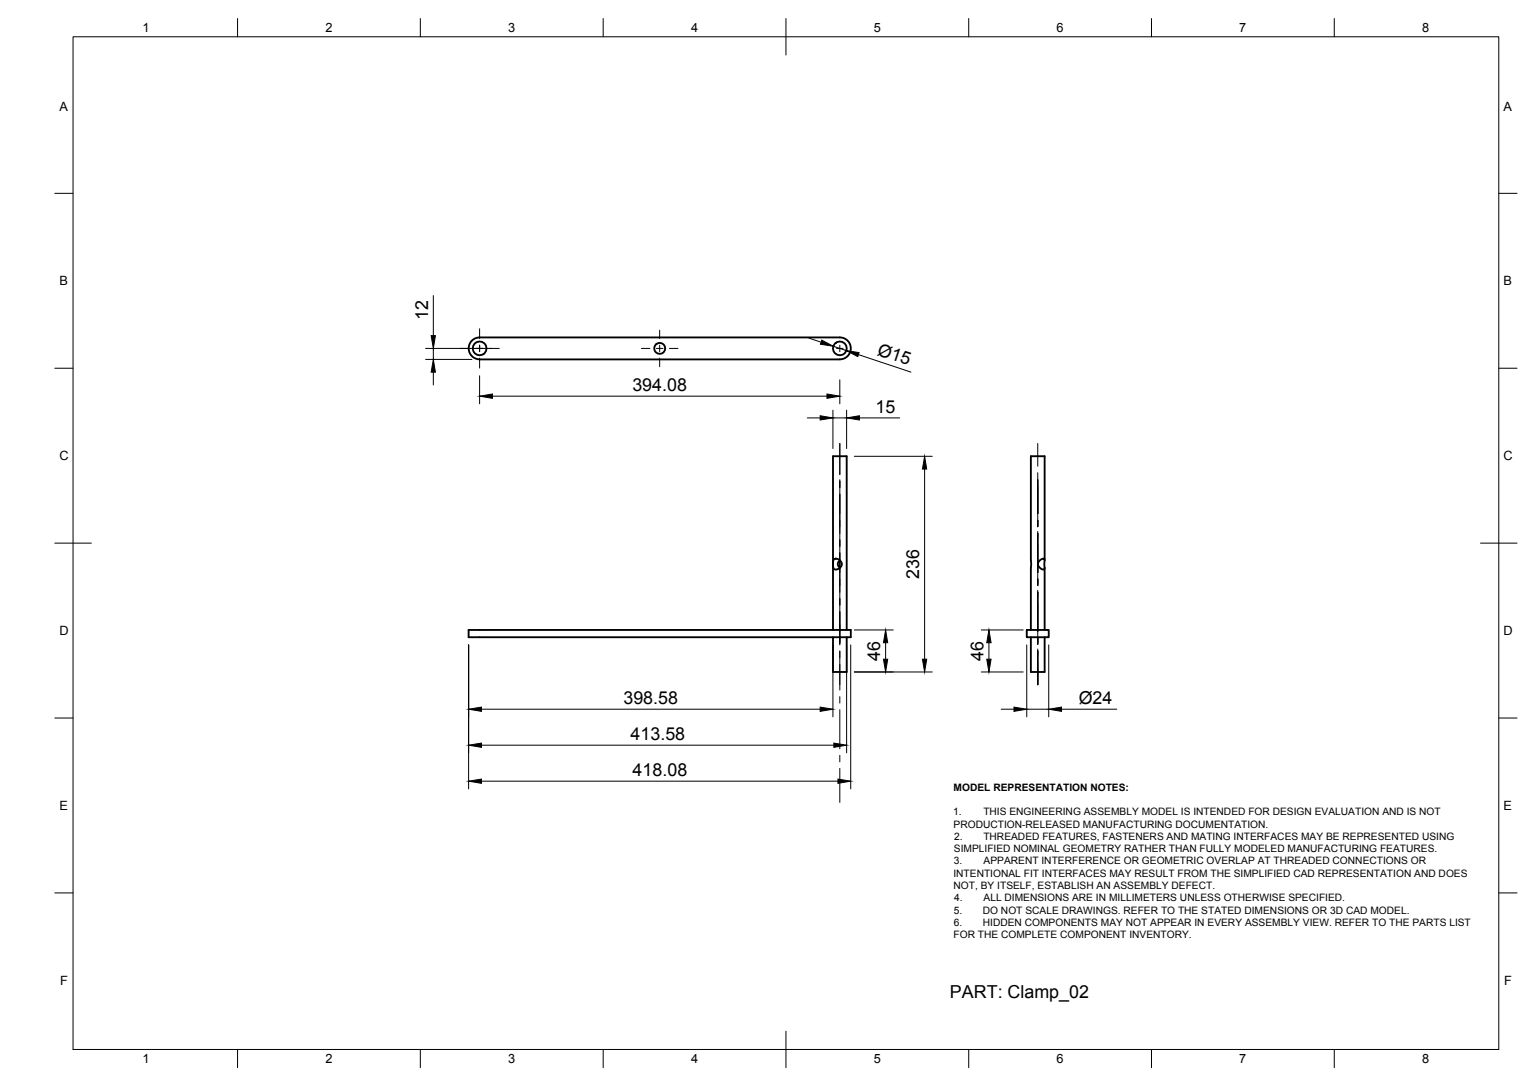
ISO-10303-21;
HEADER;
/* Generated by software containing ST-Developer
 * from STEP Tools, Inc. (www.steptools.com) 
 */

FILE_DESCRIPTION(
/* description */ (''),
/* implementation_level */ '2;1');

FILE_NAME(
/* name */ 'Clamp_02.step',
/* time_stamp */ '2026-10-05T15:35:09-07:00',
/* author */ (''),
/* organization */ (''),
/* preprocessor_version */ 'ST-DEVELOPER v20.2',
/* originating_system */ 'Autodesk Translation Framework v15.15.0.0',
/* authorisation */ '');

FILE_SCHEMA (('AUTOMOTIVE_DESIGN { 1 0 10303 214 3 1 1 }'));
ENDSEC;

DATA;
#10=MECHANICAL_DESIGN_GEOMETRIC_PRESENTATION_REPRESENTATION('',(#547),#74523);
#55=B_SPLINE_CURVE_WITH_KNOTS('',3,(#6168,#6169,#6170,#6171,#6172,#6173,
#6174,#6175,#6176,#6177,#6178,#6179),.UNSPECIFIED.,.F.,.F.,(4,2,2,2,2,4),
(0.,0.123044034193907,0.246088068387815,0.492176136775629,0.730610433663304,
0.969044730550978),.UNSPECIFIED.);
#56=B_SPLINE_CURVE_WITH_KNOTS('',3,(#6180,#6181,#6182,#6183,#6184,#6185,
#6186,#6187,#6188,#6189,#6190,#6191,#6192,#6193,#6194,#6195,#6196,#6197,
#6198,#6199,#6200,#6201,#6202,#6203,#6204,#6205,#6206,#6207,#6208,#6209,
#6210,#6211),.UNSPECIFIED.,.F.,.F.,(4,2,2,2,2,2,2,2,2,2,2,2,2,2,2,4),(0.969044730550978,
1.20747902743865,1.44591332432633,1.69200139271414,1.81504542690805,1.93808946110196,
2.06113349529586,2.18417752948977,2.43026559787759,2.66869989476526,2.90713419165293,
3.14556848854061,3.38400278542828,3.6300908538161,3.75313488801,3.87617892220391),
 .UNSPECIFIED.);
#57=B_SPLINE_CURVE_WITH_KNOTS('',3,(#6215,#6216,#6217,#6218,#6219,#6220,
#6221,#6222,#6223,#6224,#6225,#6226,#6227,#6228,#6229,#6230,#6231,#6232,
#6233,#6234,#6235,#6236),.UNSPECIFIED.,.F.,.F.,(4,2,2,2,2,2,2,2,2,2,4),
(0.969044730550978,1.20747902743865,1.44591332432633,1.69200139271414,1.81504542690805,
1.93808946110196,2.06113349529586,2.18417752948977,2.43026559787759,2.66869989476526,
2.90713419165293),.UNSPECIFIED.);
#58=B_SPLINE_CURVE_WITH_KNOTS('',3,(#6238,#6239,#6240,#6241,#6242,#6243,
#6244,#6245,#6246,#6247,#6248,#6249),.UNSPECIFIED.,.F.,.F.,(4,2,2,2,2,4),
(0.,0.123044034193907,0.246088068387815,0.492176136775629,0.730610433663304,
0.969044730550978),.UNSPECIFIED.);
#59=B_SPLINE_CURVE_WITH_KNOTS('',3,(#6250,#6251,#6252,#6253,#6254,#6255,
#6256,#6257,#6258,#6259,#6260,#6261),.UNSPECIFIED.,.F.,.F.,(4,2,2,2,2,4),
(2.90713419165293,3.14556848854061,3.38400278542828,3.6300908538161,3.75313488801,
3.87617892220391),.UNSPECIFIED.);
#529=SHAPE_REPRESENTATION_RELATIONSHIP('SRR','None',#74562,#538);
#538=ADVANCED_BREP_SHAPE_REPRESENTATION('',(#556),#74518);
#547=STYLED_ITEM('',(#74612),#556);
#556=MANIFOLD_SOLID_BREP('Body1',#4726);
#587=FACE_BOUND('',#924,.T.);
#588=FACE_BOUND('',#925,.T.);
#589=FACE_BOUND('',#926,.T.);
#590=FACE_BOUND('',#928,.T.);
#591=FACE_BOUND('',#929,.T.);
#592=FACE_BOUND('',#930,.T.);
#593=FACE_BOUND('',#934,.T.);
#643=PLANE('',#4968);
#644=PLANE('',#4972);
#645=PLANE('',#4976);
#646=PLANE('',#4978);
#647=PLANE('',#4982);
#648=PLANE('',#4985);
#746=FACE_OUTER_BOUND('',#916,.T.);
#747=FACE_OUTER_BOUND('',#917,.T.);
#748=FACE_OUTER_BOUND('',#918,.T.);
#749=FACE_OUTER_BOUND('',#919,.T.);
#750=FACE_OUTER_BOUND('',#920,.T.);
#751=FACE_OUTER_BOUND('',#921,.T.);
#752=FACE_OUTER_BOUND('',#922,.T.);
#753=FACE_OUTER_BOUND('',#923,.T.);
#754=FACE_OUTER_BOUND('',#927,.T.);
#755=FACE_OUTER_BOUND('',#931,.T.);
#756=FACE_OUTER_BOUND('',#932,.T.);
#757=FACE_OUTER_BOUND('',#933,.T.);
#758=FACE_OUTER_BOUND('',#935,.T.);
#916=EDGE_LOOP('',(#3270,#3271,#3272,#3273));
#917=EDGE_LOOP('',(#3274,#3275,#3276,#3277,#3278,#3279,#3280));
#918=EDGE_LOOP('',(#3281,#3282,#3283,#3284));
#919=EDGE_LOOP('',(#3285,#3286,#3287,#3288));
#920=EDGE_LOOP('',(#3289,#3290,#3291,#3292));
#921=EDGE_LOOP('',(#3293,#3294,#3295,#3296));
#922=EDGE_LOOP('',(#3297,#3298,#3299,#3300));
#923=EDGE_LOOP('',(#3301,#3302,#3303,#3304));
#924=EDGE_LOOP('',(#3305));
#925=EDGE_LOOP('',(#3306));
#926=EDGE_LOOP('',(#3307));
#927=EDGE_LOOP('',(#3308,#3309,#3310,#3311));
#928=EDGE_LOOP('',(#3312));
#929=EDGE_LOOP('',(#3313));
#930=EDGE_LOOP('',(#3314));
#931=EDGE_LOOP('',(#3315,#3316,#3317,#3318));
#932=EDGE_LOOP('',(#3319));
#933=EDGE_LOOP('',(#3320,#3321,#3322,#3323,#3324,#3325,#3326,#3327,#3328));
#934=EDGE_LOOP('',(#3329,#3330));
#935=EDGE_LOOP('',(#3331));
#1114=LINE('',#6163,#1311);
#1115=LINE('',#6213,#1312);
#1116=LINE('',#6266,#1313);
#1117=LINE('',#6271,#1314);
#1118=LINE('',#6273,#1315);
#1119=LINE('',#6275,#1316);
#1120=LINE('',#6276,#1317);
#1121=LINE('',#6282,#1318);
#1122=LINE('',#6285,#1319);
#1123=LINE('',#6287,#1320);
#1124=LINE('',#6288,#1321);
#1125=LINE('',#6301,#1322);
#1126=LINE('',#6304,#1323);
#1127=LINE('',#6306,#1324);
#1311=VECTOR('',#5458,6.00000000000001);
#1312=VECTOR('',#5463,6.);
#1313=VECTOR('',#5468,7.5);
#1314=VECTOR('',#5473,10.);
#1315=VECTOR('',#5474,10.);
#1316=VECTOR('',#5475,10.);
#1317=VECTOR('',#5476,10.);
#1318=VECTOR('',#5483,10.);
#1319=VECTOR('',#5486,10.);
#1320=VECTOR('',#5487,10.);
#1321=VECTOR('',#5488,10.);
#1322=VECTOR('',#5507,7.5);
#1323=VECTOR('',#5512,7.5);
#1324=VECTOR('',#5513,7.5);
#1472=CIRCLE('',#4962,6.00000000000001);
#1473=CIRCLE('',#4963,6.00000000000001);
#1474=CIRCLE('',#4966,7.5);
#1475=CIRCLE('',#4967,7.5);
#1476=CIRCLE('',#4970,12.);
#1477=CIRCLE('',#4971,12.);
#1478=CIRCLE('',#4974,12.);
#1479=CIRCLE('',#4975,12.);
#1480=CIRCLE('',#4977,7.5);
#1481=CIRCLE('',#4979,7.5);
#1482=CIRCLE('',#4981,7.5);
#1483=CIRCLE('',#4984,7.5);
#1626=VERTEX_POINT('',#6160);
#1627=VERTEX_POINT('',#6162);
#1628=VERTEX_POINT('',#6166);
#1629=VERTEX_POINT('',#6167);
#1630=VERTEX_POINT('',#6212);
#1631=VERTEX_POINT('',#6214);
#1632=VERTEX_POINT('',#6237);
#1633=VERTEX_POINT('',#6263);
#1634=VERTEX_POINT('',#6265);
#1635=VERTEX_POINT('',#6269);
#1636=VERTEX_POINT('',#6270);
#1637=VERTEX_POINT('',#6272);
#1638=VERTEX_POINT('',#6274);
#1639=VERTEX_POINT('',#6278);
#1640=VERTEX_POINT('',#6280);
#1641=VERTEX_POINT('',#6284);
#1642=VERTEX_POINT('',#6286);
#1643=VERTEX_POINT('',#6293);
#1644=VERTEX_POINT('',#6296);
#1645=VERTEX_POINT('',#6299);
#1646=VERTEX_POINT('',#6305);
#2336=EDGE_CURVE('',#1626,#1626,#1472,.T.);
#2337=EDGE_CURVE('',#1626,#1627,#1114,.T.);
#2338=EDGE_CURVE('',#1627,#1627,#1473,.T.);
#2339=EDGE_CURVE('',#1628,#1629,#55,.T.);
#2340=EDGE_CURVE('',#1629,#1628,#56,.T.);
#2341=EDGE_CURVE('',#1629,#1630,#1115,.T.);
#2342=EDGE_CURVE('',#1631,#1630,#57,.T.);
#2343=EDGE_CURVE('',#1632,#1631,#58,.T.);
#2344=EDGE_CURVE('',#1630,#1632,#59,.T.);
#2345=EDGE_CURVE('',#1633,#1633,#1474,.T.);
#2346=EDGE_CURVE('',#1633,#1634,#1116,.T.);
#2347=EDGE_CURVE('',#1634,#1634,#1475,.T.);
#2348=EDGE_CURVE('',#1635,#1636,#1117,.T.);
#2349=EDGE_CURVE('',#1636,#1637,#1118,.T.);
#2350=EDGE_CURVE('',#1638,#1637,#1119,.T.);
#2351=EDGE_CURVE('',#1635,#1638,#1120,.T.);
#2352=EDGE_CURVE('',#1639,#1635,#1476,.T.);
#2353=EDGE_CURVE('',#1640,#1638,#1477,.T.);
#2354=EDGE_CURVE('',#1639,#1640,#1121,.T.);
#2355=EDGE_CURVE('',#1641,#1639,#1122,.T.);
#2356=EDGE_CURVE('',#1642,#1640,#1123,.T.);
#2357=EDGE_CURVE('',#1641,#1642,#1124,.T.);
#2358=EDGE_CURVE('',#1636,#1641,#1478,.T.);
#2359=EDGE_CURVE('',#1637,#1642,#1479,.T.);
#2360=EDGE_CURVE('',#1643,#1643,#1480,.T.);
#2361=EDGE_CURVE('',#1644,#1644,#1481,.T.);
#2362=EDGE_CURVE('',#1645,#1645,#1482,.T.);
#2363=EDGE_CURVE('',#1645,#1644,#1125,.T.);
#2364=EDGE_CURVE('',#1643,#1630,#1126,.T.);
#2365=EDGE_CURVE('',#1631,#1646,#1127,.T.);
#2366=EDGE_CURVE('',#1646,#1646,#1483,.T.);
#3270=ORIENTED_EDGE('',*,*,#2336,.F.);
#3271=ORIENTED_EDGE('',*,*,#2337,.T.);
#3272=ORIENTED_EDGE('',*,*,#2338,.F.);
#3273=ORIENTED_EDGE('',*,*,#2337,.F.);
#3274=ORIENTED_EDGE('',*,*,#2339,.F.);
#3275=ORIENTED_EDGE('',*,*,#2340,.F.);
#3276=ORIENTED_EDGE('',*,*,#2341,.T.);
#3277=ORIENTED_EDGE('',*,*,#2342,.F.);
#3278=ORIENTED_EDGE('',*,*,#2343,.F.);
#3279=ORIENTED_EDGE('',*,*,#2344,.F.);
#3280=ORIENTED_EDGE('',*,*,#2341,.F.);
#3281=ORIENTED_EDGE('',*,*,#2345,.T.);
#3282=ORIENTED_EDGE('',*,*,#2346,.T.);
#3283=ORIENTED_EDGE('',*,*,#2347,.F.);
#3284=ORIENTED_EDGE('',*,*,#2346,.F.);
#3285=ORIENTED_EDGE('',*,*,#2348,.T.);
#3286=ORIENTED_EDGE('',*,*,#2349,.T.);
#3287=ORIENTED_EDGE('',*,*,#2350,.F.);
#3288=ORIENTED_EDGE('',*,*,#2351,.F.);
#3289=ORIENTED_EDGE('',*,*,#2352,.T.);
#3290=ORIENTED_EDGE('',*,*,#2351,.T.);
#3291=ORIENTED_EDGE('',*,*,#2353,.F.);
#3292=ORIENTED_EDGE('',*,*,#2354,.F.);
#3293=ORIENTED_EDGE('',*,*,#2355,.T.);
#3294=ORIENTED_EDGE('',*,*,#2354,.T.);
#3295=ORIENTED_EDGE('',*,*,#2356,.F.);
#3296=ORIENTED_EDGE('',*,*,#2357,.F.);
#3297=ORIENTED_EDGE('',*,*,#2358,.T.);
#3298=ORIENTED_EDGE('',*,*,#2357,.T.);
#3299=ORIENTED_EDGE('',*,*,#2359,.F.);
#3300=ORIENTED_EDGE('',*,*,#2349,.F.);
#3301=ORIENTED_EDGE('',*,*,#2359,.T.);
#3302=ORIENTED_EDGE('',*,*,#2356,.T.);
#3303=ORIENTED_EDGE('',*,*,#2353,.T.);
#3304=ORIENTED_EDGE('',*,*,#2350,.T.);
#3305=ORIENTED_EDGE('',*,*,#2336,.T.);
#3306=ORIENTED_EDGE('',*,*,#2360,.F.);
#3307=ORIENTED_EDGE('',*,*,#2347,.T.);
#3308=ORIENTED_EDGE('',*,*,#2358,.F.);
#3309=ORIENTED_EDGE('',*,*,#2348,.F.);
#3310=ORIENTED_EDGE('',*,*,#2352,.F.);
#3311=ORIENTED_EDGE('',*,*,#2355,.F.);
#3312=ORIENTED_EDGE('',*,*,#2338,.T.);
#3313=ORIENTED_EDGE('',*,*,#2361,.F.);
#3314=ORIENTED_EDGE('',*,*,#2345,.F.);
#3315=ORIENTED_EDGE('',*,*,#2362,.T.);
#3316=ORIENTED_EDGE('',*,*,#2363,.T.);
#3317=ORIENTED_EDGE('',*,*,#2361,.T.);
#3318=ORIENTED_EDGE('',*,*,#2363,.F.);
#3319=ORIENTED_EDGE('',*,*,#2362,.F.);
#3320=ORIENTED_EDGE('',*,*,#2360,.T.);
#3321=ORIENTED_EDGE('',*,*,#2364,.T.);
#3322=ORIENTED_EDGE('',*,*,#2344,.T.);
#3323=ORIENTED_EDGE('',*,*,#2343,.T.);
#3324=ORIENTED_EDGE('',*,*,#2365,.T.);
#3325=ORIENTED_EDGE('',*,*,#2366,.T.);
#3326=ORIENTED_EDGE('',*,*,#2365,.F.);
#3327=ORIENTED_EDGE('',*,*,#2342,.T.);
#3328=ORIENTED_EDGE('',*,*,#2364,.F.);
#3329=ORIENTED_EDGE('',*,*,#2339,.T.);
#3330=ORIENTED_EDGE('',*,*,#2340,.T.);
#3331=ORIENTED_EDGE('',*,*,#2366,.F.);
#4544=CYLINDRICAL_SURFACE('',#4961,6.00000000000001);
#4545=CYLINDRICAL_SURFACE('',#4964,6.);
#4546=CYLINDRICAL_SURFACE('',#4965,7.5);
#4547=CYLINDRICAL_SURFACE('',#4969,12.);
#4548=CYLINDRICAL_SURFACE('',#4973,12.);
#4549=CYLINDRICAL_SURFACE('',#4980,7.5);
#4550=CYLINDRICAL_SURFACE('',#4983,7.5);
#4642=ADVANCED_FACE('',(#746),#4544,.F.);
#4643=ADVANCED_FACE('',(#747),#4545,.F.);
#4644=ADVANCED_FACE('',(#748),#4546,.F.);
#4645=ADVANCED_FACE('',(#749),#643,.T.);
#4646=ADVANCED_FACE('',(#750),#4547,.T.);
#4647=ADVANCED_FACE('',(#751),#644,.T.);
#4648=ADVANCED_FACE('',(#752),#4548,.T.);
#4649=ADVANCED_FACE('',(#753,#587,#588,#589),#645,.T.);
#4650=ADVANCED_FACE('',(#754,#590,#591,#592),#646,.F.);
#4651=ADVANCED_FACE('',(#755),#4549,.T.);
#4652=ADVANCED_FACE('',(#756),#647,.T.);
#4653=ADVANCED_FACE('',(#757,#593),#4550,.T.);
#4654=ADVANCED_FACE('',(#758),#648,.F.);
#4726=CLOSED_SHELL('',(#4642,#4643,#4644,#4645,#4646,#4647,#4648,#4649,
#4650,#4651,#4652,#4653,#4654));
#4960=AXIS2_PLACEMENT_3D('',#6158,#5452,#5453);
#4961=AXIS2_PLACEMENT_3D('',#6159,#5454,#5455);
#4962=AXIS2_PLACEMENT_3D('',#6161,#5456,#5457);
#4963=AXIS2_PLACEMENT_3D('',#6164,#5459,#5460);
#4964=AXIS2_PLACEMENT_3D('',#6165,#5461,#5462);
#4965=AXIS2_PLACEMENT_3D('',#6262,#5464,#5465);
#4966=AXIS2_PLACEMENT_3D('',#6264,#5466,#5467);
#4967=AXIS2_PLACEMENT_3D('',#6267,#5469,#5470);
#4968=AXIS2_PLACEMENT_3D('',#6268,#5471,#5472);
#4969=AXIS2_PLACEMENT_3D('',#6277,#5477,#5478);
#4970=AXIS2_PLACEMENT_3D('',#6279,#5479,#5480);
#4971=AXIS2_PLACEMENT_3D('',#6281,#5481,#5482);
#4972=AXIS2_PLACEMENT_3D('',#6283,#5484,#5485);
#4973=AXIS2_PLACEMENT_3D('',#6289,#5489,#5490);
#4974=AXIS2_PLACEMENT_3D('',#6290,#5491,#5492);
#4975=AXIS2_PLACEMENT_3D('',#6291,#5493,#5494);
#4976=AXIS2_PLACEMENT_3D('',#6292,#5495,#5496);
#4977=AXIS2_PLACEMENT_3D('',#6294,#5497,#5498);
#4978=AXIS2_PLACEMENT_3D('',#6295,#5499,#5500);
#4979=AXIS2_PLACEMENT_3D('',#6297,#5501,#5502);
#4980=AXIS2_PLACEMENT_3D('',#6298,#5503,#5504);
#4981=AXIS2_PLACEMENT_3D('',#6300,#5505,#5506);
#4982=AXIS2_PLACEMENT_3D('',#6302,#5508,#5509);
#4983=AXIS2_PLACEMENT_3D('',#6303,#5510,#5511);
#4984=AXIS2_PLACEMENT_3D('',#6307,#5514,#5515);
#4985=AXIS2_PLACEMENT_3D('',#6308,#5516,#5517);
#5452=DIRECTION('axis',(0.,0.,1.));
#5453=DIRECTION('refdir',(1.,0.,0.));
#5454=DIRECTION('center_axis',(0.,-1.,0.));
#5455=DIRECTION('ref_axis',(1.,0.,0.));
#5456=DIRECTION('center_axis',(0.,-1.,0.));
#5457=DIRECTION('ref_axis',(1.,0.,0.));
#5458=DIRECTION('',(0.,-1.,0.));
#5459=DIRECTION('center_axis',(0.,1.,0.));
#5460=DIRECTION('ref_axis',(1.,0.,0.));
#5461=DIRECTION('center_axis',(-1.,0.,0.));
#5462=DIRECTION('ref_axis',(0.,1.,0.));
#5463=DIRECTION('',(-1.,0.,0.));
#5464=DIRECTION('center_axis',(0.,1.,0.));
#5465=DIRECTION('ref_axis',(1.,0.,0.));
#5466=DIRECTION('center_axis',(0.,-1.,0.));
#5467=DIRECTION('ref_axis',(1.,0.,0.));
#5468=DIRECTION('',(0.,1.,0.));
#5469=DIRECTION('center_axis',(0.,-1.,0.));
#5470=DIRECTION('ref_axis',(1.,0.,0.));
#5471=DIRECTION('center_axis',(-0.812015371342714,0.,0.583636048152575));
#5472=DIRECTION('ref_axis',(0.583636048152575,0.,0.812015371342714));
#5473=DIRECTION('',(0.583636048152575,0.,0.812015371342714));
#5474=DIRECTION('',(0.,1.,0.));
#5475=DIRECTION('',(0.583636048152575,0.,0.812015371342714));
#5476=DIRECTION('',(0.,1.,0.));
#5477=DIRECTION('center_axis',(0.,1.,0.));
#5478=DIRECTION('ref_axis',(0.812015371342714,0.,-0.583636048152574));
#5479=DIRECTION('center_axis',(0.,1.,0.));
#5480=DIRECTION('ref_axis',(0.812015371342714,0.,-0.583636048152574));
#5481=DIRECTION('center_axis',(0.,1.,0.));
#5482=DIRECTION('ref_axis',(0.812015371342714,0.,-0.583636048152574));
#5483=DIRECTION('',(0.,1.,0.));
#5484=DIRECTION('center_axis',(0.812015371342714,0.,-0.583636048152575));
#5485=DIRECTION('ref_axis',(-0.583636048152575,0.,-0.812015371342714));
#5486=DIRECTION('',(-0.583636048152575,0.,-0.812015371342714));
#5487=DIRECTION('',(-0.583636048152575,0.,-0.812015371342714));
#5488=DIRECTION('',(0.,1.,0.));
#5489=DIRECTION('center_axis',(0.,1.,0.));
#5490=DIRECTION('ref_axis',(-0.812015371342714,0.,0.583636048152574));
#5491=DIRECTION('center_axis',(0.,1.,0.));
#5492=DIRECTION('ref_axis',(-0.812015371342714,0.,0.583636048152574));
#5493=DIRECTION('center_axis',(0.,1.,0.));
#5494=DIRECTION('ref_axis',(-0.812015371342714,0.,0.583636048152574));
#5495=DIRECTION('center_axis',(0.,1.,0.));
#5496=DIRECTION('ref_axis',(1.,0.,0.));
#5497=DIRECTION('center_axis',(0.,1.,0.));
#5498=DIRECTION('ref_axis',(1.,0.,2.44929359829471E-16));
#5499=DIRECTION('center_axis',(0.,1.,0.));
#5500=DIRECTION('ref_axis',(1.,0.,0.));
#5501=DIRECTION('center_axis',(0.,-1.,0.));
#5502=DIRECTION('ref_axis',(1.,0.,2.44929359829471E-16));
#5503=DIRECTION('center_axis',(-3.66477378287572E-33,-1.,2.99251489117293E-17));
#5504=DIRECTION('ref_axis',(1.,3.66477378287573E-33,2.44929359829471E-16));
#5505=DIRECTION('center_axis',(3.66477378287572E-33,1.,-2.99251489117293E-17));
#5506=DIRECTION('ref_axis',(1.,3.66477378287573E-33,2.44929359829471E-16));
#5507=DIRECTION('',(3.66477378287572E-33,1.,-2.99251489117293E-17));
#5508=DIRECTION('center_axis',(-3.66477378287572E-33,-1.,2.99251489117293E-17));
#5509=DIRECTION('ref_axis',(1.,3.66477378287573E-33,2.44929359829471E-16));
#5510=DIRECTION('center_axis',(-3.66477378287572E-33,-1.,2.99251489117293E-17));
#5511=DIRECTION('ref_axis',(1.,3.66477378287573E-33,2.44929359829471E-16));
#5512=DIRECTION('',(3.66477378287572E-33,1.,-2.99251489117293E-17));
#5513=DIRECTION('',(3.66477378287572E-33,1.,-2.99251489117293E-17));
#5514=DIRECTION('center_axis',(-3.66477378287572E-33,-1.,2.99251489117293E-17));
#5515=DIRECTION('ref_axis',(1.,3.66477378287573E-33,2.44929359829471E-16));
#5516=DIRECTION('center_axis',(-3.66477378287572E-33,-1.,2.99251489117293E-17));
#5517=DIRECTION('ref_axis',(1.,3.66477378287573E-33,2.44929359829471E-16));
#6158=CARTESIAN_POINT('',(0.,0.,0.));
#6159=CARTESIAN_POINT('Origin',(60.231676812499,-95.,175.));
#6160=CARTESIAN_POINT('',(54.231676812499,-72.,175.));
#6161=CARTESIAN_POINT('Origin',(60.231676812499,-72.,175.));
#6162=CARTESIAN_POINT('',(54.231676812499,-80.,175.));
#6163=CARTESIAN_POINT('',(54.231676812499,-95.,175.));
#6164=CARTESIAN_POINT('Origin',(60.231676812499,-80.,175.));
#6165=CARTESIAN_POINT('Origin',(185.231676812499,0.,335.));
#6166=CARTESIAN_POINT('',(179.731676812499,2.46330733588707E-15,329.));
#6167=CARTESIAN_POINT('',(182.731676812499,-6.,335.));
#6168=CARTESIAN_POINT('Ctrl Pts',(179.731676812499,-1.38777878078145E-16,
329.));
#6169=CARTESIAN_POINT('Ctrl Pts',(179.731676812499,-0.410146780646358,329.));
#6170=CARTESIAN_POINT('Ctrl Pts',(179.789372806578,-0.816861849349989,329.042276815307));
#6171=CARTESIAN_POINT('Ctrl Pts',(179.994045571984,-1.60462674459781,329.204579222783));
#6172=CARTESIAN_POINT('Ctrl Pts',(180.139940991557,-1.98596758305952,329.324554046353));
#6173=CARTESIAN_POINT('Ctrl Pts',(180.642335947217,-3.07201535485507,329.786388864399));
#6174=CARTESIAN_POINT('Ctrl Pts',(181.058329790287,-3.7207625323499,330.235481158111));
#6175=CARTESIAN_POINT('Ctrl Pts',(181.763206112437,-4.74828751391861,331.26300613968));
#6176=CARTESIAN_POINT('Ctrl Pts',(182.110324034524,-5.20624497170395,331.912343858094));
#6177=CARTESIAN_POINT('Ctrl Pts',(182.596018078742,-5.8328999714949,333.382629157599));
#6178=CARTESIAN_POINT('Ctrl Pts',(182.731676812499,-6.00000000000001,334.205219010374));
#6179=CARTESIAN_POINT('Ctrl Pts',(182.731676812499,-6.00000000000001,335.));
#6180=CARTESIAN_POINT('Ctrl Pts',(182.731676812499,-6.,335.));
#6181=CARTESIAN_POINT('Ctrl Pts',(182.731676812499,-6.,335.794780989626));
#6182=CARTESIAN_POINT('Ctrl Pts',(182.596018078742,-5.8328999714949,336.617370842401));
#6183=CARTESIAN_POINT('Ctrl Pts',(182.110324034524,-5.20624497170395,338.087656141906));
#6184=CARTESIAN_POINT('Ctrl Pts',(181.763206112437,-4.74828751391861,338.73699386032));
#6185=CARTESIAN_POINT('Ctrl Pts',(181.058329790287,-3.7207625323499,339.764518841889));
#6186=CARTESIAN_POINT('Ctrl Pts',(180.642335947217,-3.07201535485507,340.213611135601));
#6187=CARTESIAN_POINT('Ctrl Pts',(180.139940991557,-1.98596758305952,340.675445953647));
#6188=CARTESIAN_POINT('Ctrl Pts',(179.994045571984,-1.60462674459781,340.795420777217));
#6189=CARTESIAN_POINT('Ctrl Pts',(179.789372806578,-0.816861849349989,340.957723184693));
#6190=CARTESIAN_POINT('Ctrl Pts',(179.731676812499,-0.410146780646358,341.));
#6191=CARTESIAN_POINT('Ctrl Pts',(179.731676812499,0.410146780646357,341.));
#6192=CARTESIAN_POINT('Ctrl Pts',(179.789372806578,0.816861849350014,340.957723184693));
#6193=CARTESIAN_POINT('Ctrl Pts',(179.994045571984,1.60462674459784,340.795420777217));
#6194=CARTESIAN_POINT('Ctrl Pts',(180.139940991557,1.9859675830595,340.675445953647));
#6195=CARTESIAN_POINT('Ctrl Pts',(180.642335947218,3.07201535485506,340.213611135601));
#6196=CARTESIAN_POINT('Ctrl Pts',(181.058329790287,3.7207625323499,339.764518841889));
#6197=CARTESIAN_POINT('Ctrl Pts',(181.763206112437,4.74828751391861,338.73699386032));
#6198=CARTESIAN_POINT('Ctrl Pts',(182.110324034524,5.20624497170395,338.087656141906));
#6199=CARTESIAN_POINT('Ctrl Pts',(182.596018078742,5.8328999714949,336.617370842401));
#6200=CARTESIAN_POINT('Ctrl Pts',(182.731676812499,6.,335.794780989626));
#6201=CARTESIAN_POINT('Ctrl Pts',(182.731676812499,6.,334.205219010374));
#6202=CARTESIAN_POINT('Ctrl Pts',(182.596018078742,5.8328999714949,333.382629157599));
#6203=CARTESIAN_POINT('Ctrl Pts',(182.110324034524,5.20624497170395,331.912343858094));
#6204=CARTESIAN_POINT('Ctrl Pts',(181.763206112437,4.74828751391861,331.26300613968));
#6205=CARTESIAN_POINT('Ctrl Pts',(181.058329790287,3.7207625323499,330.235481158111));
#6206=CARTESIAN_POINT('Ctrl Pts',(180.642335947218,3.07201535485506,329.786388864399));
#6207=CARTESIAN_POINT('Ctrl Pts',(180.139940991557,1.9859675830595,329.324554046353));
#6208=CARTESIAN_POINT('Ctrl Pts',(179.994045571984,1.60462674459784,329.204579222783));
#6209=CARTESIAN_POINT('Ctrl Pts',(179.789372806578,0.816861849350014,329.042276815307));
#6210=CARTESIAN_POINT('Ctrl Pts',(179.731676812499,0.410146780646354,329.));
#6211=CARTESIAN_POINT('Ctrl Pts',(179.731676812499,-2.67147415300428E-15,
329.));
#6212=CARTESIAN_POINT('',(167.731676812499,-6.,335.));
#6213=CARTESIAN_POINT('',(185.231676812499,-6.,335.));
#6214=CARTESIAN_POINT('',(167.731676812499,6.,335.));
#6215=CARTESIAN_POINT('Ctrl Pts',(167.731676812499,6.,335.));
#6216=CARTESIAN_POINT('Ctrl Pts',(167.731676812499,6.,335.794780989625));
#6217=CARTESIAN_POINT('Ctrl Pts',(167.867335546256,5.8328999714949,336.617370842401));
#6218=CARTESIAN_POINT('Ctrl Pts',(168.353029590474,5.20624497170395,338.087656141906));
#6219=CARTESIAN_POINT('Ctrl Pts',(168.700147512561,4.74828751391861,338.73699386032));
#6220=CARTESIAN_POINT('Ctrl Pts',(169.405023834711,3.7207625323499,339.764518841889));
#6221=CARTESIAN_POINT('Ctrl Pts',(169.821017677781,3.07201535485507,340.213611135601));
#6222=CARTESIAN_POINT('Ctrl Pts',(170.323412633441,1.98596758305952,340.675445953647));
#6223=CARTESIAN_POINT('Ctrl Pts',(170.469308053014,1.60462674459781,340.795420777217));
#6224=CARTESIAN_POINT('Ctrl Pts',(170.67398081842,0.81686184934999,340.957723184693));
#6225=CARTESIAN_POINT('Ctrl Pts',(170.731676812499,0.410146780646358,341.));
#6226=CARTESIAN_POINT('Ctrl Pts',(170.731676812499,-0.410146780646357,341.));
#6227=CARTESIAN_POINT('Ctrl Pts',(170.67398081842,-0.816861849349986,340.957723184693));
#6228=CARTESIAN_POINT('Ctrl Pts',(170.469308053014,-1.60462674459781,340.795420777217));
#6229=CARTESIAN_POINT('Ctrl Pts',(170.323412633441,-1.98596758305952,340.675445953647));
#6230=CARTESIAN_POINT('Ctrl Pts',(169.821017677781,-3.07201535485507,340.213611135601));
#6231=CARTESIAN_POINT('Ctrl Pts',(169.405023834711,-3.7207625323499,339.764518841889));
#6232=CARTESIAN_POINT('Ctrl Pts',(168.700147512561,-4.74828751391861,338.73699386032));
#6233=CARTESIAN_POINT('Ctrl Pts',(168.353029590474,-5.20624497170395,338.087656141906));
#6234=CARTESIAN_POINT('Ctrl Pts',(167.867335546256,-5.8328999714949,336.617370842401));
#6235=CARTESIAN_POINT('Ctrl Pts',(167.731676812499,-6.,335.794780989626));
#6236=CARTESIAN_POINT('Ctrl Pts',(167.731676812499,-6.,335.));
#6237=CARTESIAN_POINT('',(170.731676812499,5.89805981832114E-16,329.));
#6238=CARTESIAN_POINT('Ctrl Pts',(170.731676812499,1.2490009027033E-15,
329.));
#6239=CARTESIAN_POINT('Ctrl Pts',(170.731676812499,0.410146780646359,329.));
#6240=CARTESIAN_POINT('Ctrl Pts',(170.67398081842,0.816861849349989,329.042276815307));
#6241=CARTESIAN_POINT('Ctrl Pts',(170.469308053014,1.60462674459781,329.204579222783));
#6242=CARTESIAN_POINT('Ctrl Pts',(170.323412633441,1.98596758305952,329.324554046353));
#6243=CARTESIAN_POINT('Ctrl Pts',(169.821017677781,3.07201535485507,329.786388864399));
#6244=CARTESIAN_POINT('Ctrl Pts',(169.405023834711,3.7207625323499,330.235481158111));
#6245=CARTESIAN_POINT('Ctrl Pts',(168.700147512561,4.74828751391861,331.26300613968));
#6246=CARTESIAN_POINT('Ctrl Pts',(168.353029590474,5.20624497170395,331.912343858094));
#6247=CARTESIAN_POINT('Ctrl Pts',(167.867335546256,5.8328999714949,333.382629157599));
#6248=CARTESIAN_POINT('Ctrl Pts',(167.731676812499,6.,334.205219010374));
#6249=CARTESIAN_POINT('Ctrl Pts',(167.731676812499,6.,335.));
#6250=CARTESIAN_POINT('Ctrl Pts',(167.731676812499,-6.,335.));
#6251=CARTESIAN_POINT('Ctrl Pts',(167.731676812499,-6.,334.205219010374));
#6252=CARTESIAN_POINT('Ctrl Pts',(167.867335546256,-5.8328999714949,333.382629157599));
#6253=CARTESIAN_POINT('Ctrl Pts',(168.353029590474,-5.20624497170395,331.912343858094));
#6254=CARTESIAN_POINT('Ctrl Pts',(168.700147512561,-4.74828751391861,331.26300613968));
#6255=CARTESIAN_POINT('Ctrl Pts',(169.405023834711,-3.7207625323499,330.235481158111));
#6256=CARTESIAN_POINT('Ctrl Pts',(169.821017677781,-3.07201535485506,329.786388864399));
#6257=CARTESIAN_POINT('Ctrl Pts',(170.323412633441,-1.98596758305952,329.324554046353));
#6258=CARTESIAN_POINT('Ctrl Pts',(170.469308053014,-1.60462674459781,329.204579222783));
#6259=CARTESIAN_POINT('Ctrl Pts',(170.67398081842,-0.816861849349986,329.042276815307));
#6260=CARTESIAN_POINT('Ctrl Pts',(170.731676812499,-0.410146780646357,329.));
#6261=CARTESIAN_POINT('Ctrl Pts',(170.731676812499,-1.79550893470375E-16,
329.));
#6262=CARTESIAN_POINT('Origin',(-54.7683231875009,-80.,15.));
#6263=CARTESIAN_POINT('',(-62.2683231875009,-80.,15.));
#6264=CARTESIAN_POINT('Origin',(-54.7683231875009,-80.,15.));
#6265=CARTESIAN_POINT('',(-62.2683231875009,-72.,15.));
#6266=CARTESIAN_POINT('',(-62.2683231875009,-80.,15.));
#6267=CARTESIAN_POINT('Origin',(-54.7683231875009,-72.,15.));
#6268=CARTESIAN_POINT('Origin',(-64.5125076436135,-80.,22.0036325778309));
#6269=CARTESIAN_POINT('',(-64.5125076436135,-80.,22.0036325778309));
#6270=CARTESIAN_POINT('',(165.487492356386,-80.,342.003632577831));
#6271=CARTESIAN_POINT('',(-64.5125076436135,-80.,22.0036325778309));
#6272=CARTESIAN_POINT('',(165.487492356386,-72.,342.003632577831));
#6273=CARTESIAN_POINT('',(165.487492356386,-80.,342.003632577831));
#6274=CARTESIAN_POINT('',(-64.5125076436135,-72.,22.0036325778309));
#6275=CARTESIAN_POINT('',(-64.5125076436135,-72.,22.0036325778309));
#6276=CARTESIAN_POINT('',(-64.5125076436135,-80.,22.0036325778309));
#6277=CARTESIAN_POINT('Origin',(-54.7683231875009,-80.,15.));
#6278=CARTESIAN_POINT('',(-45.0241387313884,-80.,7.99636742216912));
#6279=CARTESIAN_POINT('Origin',(-54.7683231875009,-80.,15.));
#6280=CARTESIAN_POINT('',(-45.0241387313884,-72.,7.99636742216912));
#6281=CARTESIAN_POINT('Origin',(-54.7683231875009,-72.,15.));
#6282=CARTESIAN_POINT('',(-45.0241387313884,-80.,7.99636742216912));
#6283=CARTESIAN_POINT('Origin',(184.975861268612,-80.,327.996367422169));
#6284=CARTESIAN_POINT('',(184.975861268612,-80.,327.996367422169));
#6285=CARTESIAN_POINT('',(184.975861268612,-80.,327.996367422169));
#6286=CARTESIAN_POINT('',(184.975861268612,-72.,327.996367422169));
#6287=CARTESIAN_POINT('',(184.975861268612,-72.,327.996367422169));
#6288=CARTESIAN_POINT('',(184.975861268612,-80.,327.996367422169));
#6289=CARTESIAN_POINT('Origin',(175.231676812499,-80.,335.));
#6290=CARTESIAN_POINT('Origin',(175.231676812499,-80.,335.));
#6291=CARTESIAN_POINT('Origin',(175.231676812499,-72.,335.));
#6292=CARTESIAN_POINT('Origin',(60.231676812499,-72.,175.));
#6293=CARTESIAN_POINT('',(167.731676812499,-72.,335.));
#6294=CARTESIAN_POINT('Origin',(175.231676812499,-72.,335.));
#6295=CARTESIAN_POINT('Origin',(60.231676812499,-80.,175.));
#6296=CARTESIAN_POINT('',(167.731676812499,-80.,335.));
#6297=CARTESIAN_POINT('Origin',(175.231676812499,-80.,335.));
#6298=CARTESIAN_POINT('Origin',(175.231676812499,4.78802382587669E-15,335.));
#6299=CARTESIAN_POINT('',(167.731676812499,-118.,335.));
#6300=CARTESIAN_POINT('Origin',(175.231676812499,-118.,335.));
#6301=CARTESIAN_POINT('',(167.731676812499,4.78802382587669E-15,335.));
#6302=CARTESIAN_POINT('Origin',(175.231676812499,-118.,335.));
#6303=CARTESIAN_POINT('Origin',(175.231676812499,4.78802382587669E-15,335.));
#6304=CARTESIAN_POINT('',(167.731676812499,4.78802382587669E-15,335.));
#6305=CARTESIAN_POINT('',(167.731676812499,118.,335.));
#6306=CARTESIAN_POINT('',(167.731676812499,4.78802382587669E-15,335.));
#6307=CARTESIAN_POINT('Origin',(175.231676812499,118.,335.));
#6308=CARTESIAN_POINT('Origin',(175.231676812499,118.,335.));
#74507=UNCERTAINTY_MEASURE_WITH_UNIT(LENGTH_MEASURE(0.01),#74524,
'DISTANCE_ACCURACY_VALUE',
'Maximum model space distance between geometric entities at asserted c
onnectivities');
#74512=UNCERTAINTY_MEASURE_WITH_UNIT(LENGTH_MEASURE(0.01),#74524,
'DISTANCE_ACCURACY_VALUE',
'Maximum model space distance between geometric entities at asserted c
onnectivities');
#74518=(
GEOMETRIC_REPRESENTATION_CONTEXT(3)
GLOBAL_UNCERTAINTY_ASSIGNED_CONTEXT((#74507))
GLOBAL_UNIT_ASSIGNED_CONTEXT((#74524,#74526,#74527))
REPRESENTATION_CONTEXT('','3D')
);
#74523=(
GEOMETRIC_REPRESENTATION_CONTEXT(3)
GLOBAL_UNCERTAINTY_ASSIGNED_CONTEXT((#74512))
GLOBAL_UNIT_ASSIGNED_CONTEXT((#74524,#74526,#74527))
REPRESENTATION_CONTEXT('','3D')
);
#74524=(
LENGTH_UNIT()
NAMED_UNIT(*)
SI_UNIT(.MILLI.,.METRE.)
);
#74526=(
NAMED_UNIT(*)
PLANE_ANGLE_UNIT()
SI_UNIT($,.RADIAN.)
);
#74527=(
NAMED_UNIT(*)
SI_UNIT($,.STERADIAN.)
SOLID_ANGLE_UNIT()
);
#74533=SHAPE_DEFINITION_REPRESENTATION(#74543,#74562);
#74543=PRODUCT_DEFINITION_SHAPE('',$,#74573);
#74562=SHAPE_REPRESENTATION('',(#4960),#74518);
#74567=PRODUCT_DEFINITION_CONTEXT('part definition',#74599,'design');
#74573=PRODUCT_DEFINITION('Clamp_02','Clamp_02',#74583,#74567);
#74583=PRODUCT_DEFINITION_FORMATION('',$,#74606);
#74599=APPLICATION_CONTEXT(
'Core Data for Automotive Mechanical Design Process');
#74600=PRODUCT_CONTEXT('part definition',#74599,'mechanical');
#74606=PRODUCT('Clamp_02','Clamp_02',$,(#74600));
#74612=PRESENTATION_STYLE_ASSIGNMENT((#74615));
#74615=SURFACE_STYLE_USAGE(.BOTH.,#74618);
#74618=SURFACE_SIDE_STYLE('',(#74621));
#74621=SURFACE_STYLE_FILL_AREA(#74624);
#74624=FILL_AREA_STYLE('Opaque(215,0,0)',(#74627));
#74627=FILL_AREA_STYLE_COLOUR('Opaque(215,0,0)',#74630);
#74630=COLOUR_RGB('Opaque(215,0,0)', 0.09019608, 0.27058824, 0.51372549);
ENDSEC;
END-ISO-10303-21;
